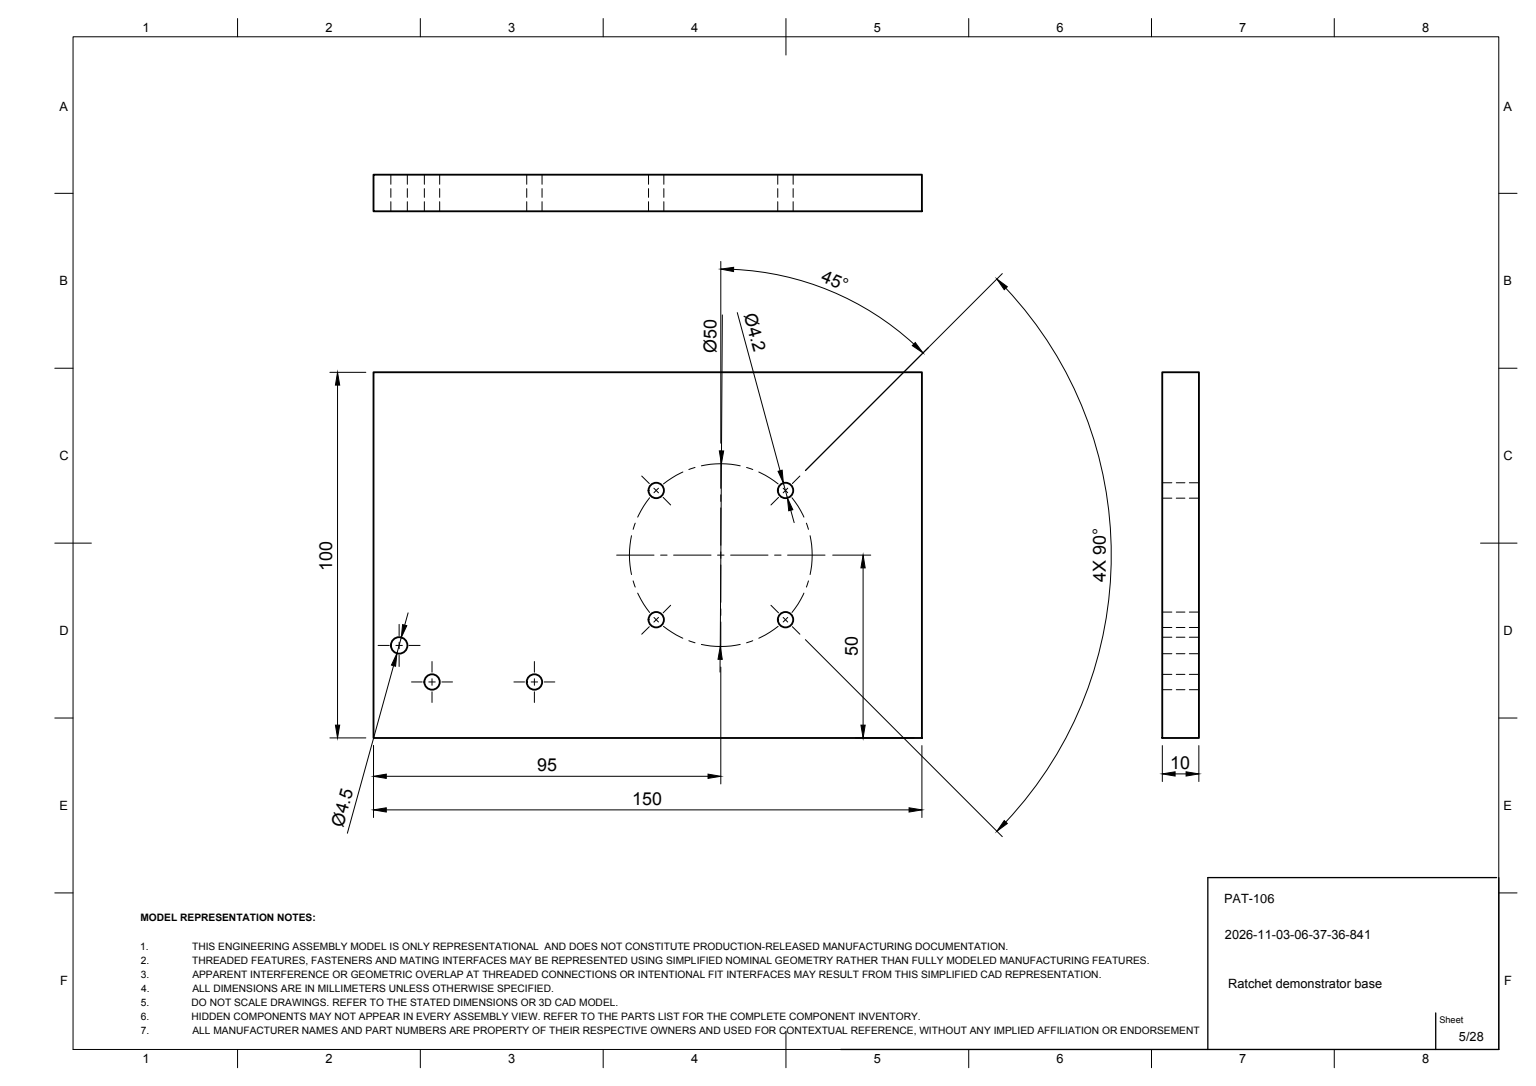
ISO-10303-21;
HEADER;
/* Generated by software containing ST-Developer
 * from STEP Tools, Inc. (www.steptools.com) 
 */

FILE_DESCRIPTION(
/* description */ ('Torsion-spring ratchet demonstrator'),
/* implementation_level */ '2;1');

FILE_NAME(
/* name */ 'Ratchet demonstrator base.step',
/* time_stamp */ '2026-10-29T17:29:17-07:00',
/* author */ (''),
/* organization */ (''),
/* preprocessor_version */ 'ST-DEVELOPER v20.2',
/* originating_system */ 'Autodesk Translation Framework v15.17.0.0',
/* authorisation */ '');

FILE_SCHEMA (('AUTOMOTIVE_DESIGN { 1 0 10303 214 3 1 1 }'));
ENDSEC;

DATA;
#10=MECHANICAL_DESIGN_GEOMETRIC_PRESENTATION_REPRESENTATION('',(#283),#11258);
#235=SHAPE_REPRESENTATION_RELATIONSHIP('SRR','None',#11361,#259);
#259=ADVANCED_BREP_SHAPE_REPRESENTATION('',(#315),#11231);
#283=STYLED_ITEM('',(#11563),#315);
#315=MANIFOLD_SOLID_BREP('Body1',#5154);
#345=FACE_BOUND('',#940,.T.);
#346=FACE_BOUND('',#941,.T.);
#347=FACE_BOUND('',#942,.T.);
#348=FACE_BOUND('',#943,.T.);
#349=FACE_BOUND('',#944,.T.);
#350=FACE_BOUND('',#945,.T.);
#351=FACE_BOUND('',#946,.T.);
#352=FACE_BOUND('',#948,.T.);
#353=FACE_BOUND('',#949,.T.);
#354=FACE_BOUND('',#950,.T.);
#355=FACE_BOUND('',#951,.T.);
#356=FACE_BOUND('',#952,.T.);
#357=FACE_BOUND('',#953,.T.);
#358=FACE_BOUND('',#954,.T.);
#437=PLANE('',#5477);
#438=PLANE('',#5478);
#439=PLANE('',#5479);
#440=PLANE('',#5480);
#441=PLANE('',#5481);
#442=PLANE('',#5482);
#623=FACE_OUTER_BOUND('',#928,.T.);
#624=FACE_OUTER_BOUND('',#929,.T.);
#625=FACE_OUTER_BOUND('',#930,.T.);
#626=FACE_OUTER_BOUND('',#931,.T.);
#627=FACE_OUTER_BOUND('',#932,.T.);
#628=FACE_OUTER_BOUND('',#933,.T.);
#629=FACE_OUTER_BOUND('',#934,.T.);
#630=FACE_OUTER_BOUND('',#935,.T.);
#631=FACE_OUTER_BOUND('',#936,.T.);
#632=FACE_OUTER_BOUND('',#937,.T.);
#633=FACE_OUTER_BOUND('',#938,.T.);
#634=FACE_OUTER_BOUND('',#939,.T.);
#635=FACE_OUTER_BOUND('',#947,.T.);
#928=EDGE_LOOP('',(#3442,#3443,#3444,#3445));
#929=EDGE_LOOP('',(#3446,#3447,#3448,#3449));
#930=EDGE_LOOP('',(#3450,#3451,#3452,#3453));
#931=EDGE_LOOP('',(#3454,#3455,#3456,#3457));
#932=EDGE_LOOP('',(#3458,#3459,#3460,#3461));
#933=EDGE_LOOP('',(#3462,#3463,#3464,#3465));
#934=EDGE_LOOP('',(#3466,#3467,#3468,#3469));
#935=EDGE_LOOP('',(#3470,#3471,#3472,#3473));
#936=EDGE_LOOP('',(#3474,#3475,#3476,#3477));
#937=EDGE_LOOP('',(#3478,#3479,#3480,#3481));
#938=EDGE_LOOP('',(#3482,#3483,#3484,#3485));
#939=EDGE_LOOP('',(#3486,#3487,#3488,#3489));
#940=EDGE_LOOP('',(#3490));
#941=EDGE_LOOP('',(#3491));
#942=EDGE_LOOP('',(#3492));
#943=EDGE_LOOP('',(#3493));
#944=EDGE_LOOP('',(#3494));
#945=EDGE_LOOP('',(#3495));
#946=EDGE_LOOP('',(#3496));
#947=EDGE_LOOP('',(#3497,#3498,#3499,#3500));
#948=EDGE_LOOP('',(#3501));
#949=EDGE_LOOP('',(#3502));
#950=EDGE_LOOP('',(#3503));
#951=EDGE_LOOP('',(#3504));
#952=EDGE_LOOP('',(#3505));
#953=EDGE_LOOP('',(#3506));
#954=EDGE_LOOP('',(#3507));
#1325=LINE('',#7682,#1708);
#1326=LINE('',#7688,#1709);
#1327=LINE('',#7694,#1710);
#1328=LINE('',#7700,#1711);
#1329=LINE('',#7706,#1712);
#1330=LINE('',#7712,#1713);
#1331=LINE('',#7718,#1714);
#1332=LINE('',#7723,#1715);
#1333=LINE('',#7725,#1716);
#1334=LINE('',#7727,#1717);
#1335=LINE('',#7728,#1718);
#1336=LINE('',#7731,#1719);
#1337=LINE('',#7733,#1720);
#1338=LINE('',#7734,#1721);
#1339=LINE('',#7737,#1722);
#1340=LINE('',#7739,#1723);
#1341=LINE('',#7740,#1724);
#1342=LINE('',#7742,#1725);
#1343=LINE('',#7743,#1726);
#1708=VECTOR('',#6076,0.225);
#1709=VECTOR('',#6083,0.210000000000001);
#1710=VECTOR('',#6090,0.21);
#1711=VECTOR('',#6097,0.21);
#1712=VECTOR('',#6104,0.21);
#1713=VECTOR('',#6111,0.21);
#1714=VECTOR('',#6118,0.21);
#1715=VECTOR('',#6123,1.);
#1716=VECTOR('',#6124,1.);
#1717=VECTOR('',#6125,1.);
#1718=VECTOR('',#6126,1.);
#1719=VECTOR('',#6129,1.);
#1720=VECTOR('',#6130,1.);
#1721=VECTOR('',#6131,1.);
#1722=VECTOR('',#6134,1.);
#1723=VECTOR('',#6135,1.);
#1724=VECTOR('',#6136,1.);
#1725=VECTOR('',#6139,1.);
#1726=VECTOR('',#6140,1.);
#2091=CIRCLE('',#5457,0.225);
#2092=CIRCLE('',#5458,0.225);
#2093=CIRCLE('',#5460,0.210000000000001);
#2094=CIRCLE('',#5461,0.210000000000001);
#2095=CIRCLE('',#5463,0.21);
#2096=CIRCLE('',#5464,0.21);
#2097=CIRCLE('',#5466,0.21);
#2098=CIRCLE('',#5467,0.21);
#2099=CIRCLE('',#5469,0.21);
#2100=CIRCLE('',#5470,0.21);
#2101=CIRCLE('',#5472,0.21);
#2102=CIRCLE('',#5473,0.21);
#2103=CIRCLE('',#5475,0.21);
#2104=CIRCLE('',#5476,0.21);
#2335=VERTEX_POINT('',#7679);
#2336=VERTEX_POINT('',#7681);
#2337=VERTEX_POINT('',#7685);
#2338=VERTEX_POINT('',#7687);
#2339=VERTEX_POINT('',#7691);
#2340=VERTEX_POINT('',#7693);
#2341=VERTEX_POINT('',#7697);
#2342=VERTEX_POINT('',#7699);
#2343=VERTEX_POINT('',#7703);
#2344=VERTEX_POINT('',#7705);
#2345=VERTEX_POINT('',#7709);
#2346=VERTEX_POINT('',#7711);
#2347=VERTEX_POINT('',#7715);
#2348=VERTEX_POINT('',#7717);
#2349=VERTEX_POINT('',#7721);
#2350=VERTEX_POINT('',#7722);
#2351=VERTEX_POINT('',#7724);
#2352=VERTEX_POINT('',#7726);
#2353=VERTEX_POINT('',#7730);
#2354=VERTEX_POINT('',#7732);
#2355=VERTEX_POINT('',#7736);
#2356=VERTEX_POINT('',#7738);
#2781=EDGE_CURVE('',#2335,#2335,#2091,.T.);
#2782=EDGE_CURVE('',#2335,#2336,#1325,.T.);
#2783=EDGE_CURVE('',#2336,#2336,#2092,.T.);
#2784=EDGE_CURVE('',#2337,#2337,#2093,.T.);
#2785=EDGE_CURVE('',#2337,#2338,#1326,.T.);
#2786=EDGE_CURVE('',#2338,#2338,#2094,.T.);
#2787=EDGE_CURVE('',#2339,#2339,#2095,.T.);
#2788=EDGE_CURVE('',#2339,#2340,#1327,.T.);
#2789=EDGE_CURVE('',#2340,#2340,#2096,.T.);
#2790=EDGE_CURVE('',#2341,#2341,#2097,.T.);
#2791=EDGE_CURVE('',#2341,#2342,#1328,.T.);
#2792=EDGE_CURVE('',#2342,#2342,#2098,.T.);
#2793=EDGE_CURVE('',#2343,#2343,#2099,.T.);
#2794=EDGE_CURVE('',#2343,#2344,#1329,.T.);
#2795=EDGE_CURVE('',#2344,#2344,#2100,.T.);
#2796=EDGE_CURVE('',#2345,#2345,#2101,.T.);
#2797=EDGE_CURVE('',#2345,#2346,#1330,.T.);
#2798=EDGE_CURVE('',#2346,#2346,#2102,.T.);
#2799=EDGE_CURVE('',#2347,#2347,#2103,.T.);
#2800=EDGE_CURVE('',#2347,#2348,#1331,.T.);
#2801=EDGE_CURVE('',#2348,#2348,#2104,.T.);
#2802=EDGE_CURVE('',#2349,#2350,#1332,.T.);
#2803=EDGE_CURVE('',#2350,#2351,#1333,.T.);
#2804=EDGE_CURVE('',#2352,#2351,#1334,.T.);
#2805=EDGE_CURVE('',#2349,#2352,#1335,.T.);
#2806=EDGE_CURVE('',#2353,#2349,#1336,.T.);
#2807=EDGE_CURVE('',#2354,#2352,#1337,.T.);
#2808=EDGE_CURVE('',#2353,#2354,#1338,.T.);
#2809=EDGE_CURVE('',#2355,#2353,#1339,.T.);
#2810=EDGE_CURVE('',#2356,#2354,#1340,.T.);
#2811=EDGE_CURVE('',#2355,#2356,#1341,.T.);
#2812=EDGE_CURVE('',#2350,#2355,#1342,.T.);
#2813=EDGE_CURVE('',#2351,#2356,#1343,.T.);
#3442=ORIENTED_EDGE('',*,*,#2781,.F.);
#3443=ORIENTED_EDGE('',*,*,#2782,.T.);
#3444=ORIENTED_EDGE('',*,*,#2783,.F.);
#3445=ORIENTED_EDGE('',*,*,#2782,.F.);
#3446=ORIENTED_EDGE('',*,*,#2784,.F.);
#3447=ORIENTED_EDGE('',*,*,#2785,.T.);
#3448=ORIENTED_EDGE('',*,*,#2786,.F.);
#3449=ORIENTED_EDGE('',*,*,#2785,.F.);
#3450=ORIENTED_EDGE('',*,*,#2787,.F.);
#3451=ORIENTED_EDGE('',*,*,#2788,.T.);
#3452=ORIENTED_EDGE('',*,*,#2789,.F.);
#3453=ORIENTED_EDGE('',*,*,#2788,.F.);
#3454=ORIENTED_EDGE('',*,*,#2790,.F.);
#3455=ORIENTED_EDGE('',*,*,#2791,.T.);
#3456=ORIENTED_EDGE('',*,*,#2792,.F.);
#3457=ORIENTED_EDGE('',*,*,#2791,.F.);
#3458=ORIENTED_EDGE('',*,*,#2793,.F.);
#3459=ORIENTED_EDGE('',*,*,#2794,.T.);
#3460=ORIENTED_EDGE('',*,*,#2795,.F.);
#3461=ORIENTED_EDGE('',*,*,#2794,.F.);
#3462=ORIENTED_EDGE('',*,*,#2796,.F.);
#3463=ORIENTED_EDGE('',*,*,#2797,.T.);
#3464=ORIENTED_EDGE('',*,*,#2798,.F.);
#3465=ORIENTED_EDGE('',*,*,#2797,.F.);
#3466=ORIENTED_EDGE('',*,*,#2799,.F.);
#3467=ORIENTED_EDGE('',*,*,#2800,.T.);
#3468=ORIENTED_EDGE('',*,*,#2801,.F.);
#3469=ORIENTED_EDGE('',*,*,#2800,.F.);
#3470=ORIENTED_EDGE('',*,*,#2802,.T.);
#3471=ORIENTED_EDGE('',*,*,#2803,.T.);
#3472=ORIENTED_EDGE('',*,*,#2804,.F.);
#3473=ORIENTED_EDGE('',*,*,#2805,.F.);
#3474=ORIENTED_EDGE('',*,*,#2806,.T.);
#3475=ORIENTED_EDGE('',*,*,#2805,.T.);
#3476=ORIENTED_EDGE('',*,*,#2807,.F.);
#3477=ORIENTED_EDGE('',*,*,#2808,.F.);
#3478=ORIENTED_EDGE('',*,*,#2809,.T.);
#3479=ORIENTED_EDGE('',*,*,#2808,.T.);
#3480=ORIENTED_EDGE('',*,*,#2810,.F.);
#3481=ORIENTED_EDGE('',*,*,#2811,.F.);
#3482=ORIENTED_EDGE('',*,*,#2812,.T.);
#3483=ORIENTED_EDGE('',*,*,#2811,.T.);
#3484=ORIENTED_EDGE('',*,*,#2813,.F.);
#3485=ORIENTED_EDGE('',*,*,#2803,.F.);
#3486=ORIENTED_EDGE('',*,*,#2813,.T.);
#3487=ORIENTED_EDGE('',*,*,#2810,.T.);
#3488=ORIENTED_EDGE('',*,*,#2807,.T.);
#3489=ORIENTED_EDGE('',*,*,#2804,.T.);
#3490=ORIENTED_EDGE('',*,*,#2783,.T.);
#3491=ORIENTED_EDGE('',*,*,#2786,.T.);
#3492=ORIENTED_EDGE('',*,*,#2789,.T.);
#3493=ORIENTED_EDGE('',*,*,#2792,.T.);
#3494=ORIENTED_EDGE('',*,*,#2795,.T.);
#3495=ORIENTED_EDGE('',*,*,#2798,.T.);
#3496=ORIENTED_EDGE('',*,*,#2801,.T.);
#3497=ORIENTED_EDGE('',*,*,#2812,.F.);
#3498=ORIENTED_EDGE('',*,*,#2802,.F.);
#3499=ORIENTED_EDGE('',*,*,#2806,.F.);
#3500=ORIENTED_EDGE('',*,*,#2809,.F.);
#3501=ORIENTED_EDGE('',*,*,#2781,.T.);
#3502=ORIENTED_EDGE('',*,*,#2784,.T.);
#3503=ORIENTED_EDGE('',*,*,#2787,.T.);
#3504=ORIENTED_EDGE('',*,*,#2790,.T.);
#3505=ORIENTED_EDGE('',*,*,#2793,.T.);
#3506=ORIENTED_EDGE('',*,*,#2796,.T.);
#3507=ORIENTED_EDGE('',*,*,#2799,.T.);
#4764=CYLINDRICAL_SURFACE('',#5456,0.225);
#4765=CYLINDRICAL_SURFACE('',#5459,0.210000000000001);
#4766=CYLINDRICAL_SURFACE('',#5462,0.21);
#4767=CYLINDRICAL_SURFACE('',#5465,0.21);
#4768=CYLINDRICAL_SURFACE('',#5468,0.21);
#4769=CYLINDRICAL_SURFACE('',#5471,0.21);
#4770=CYLINDRICAL_SURFACE('',#5474,0.21);
#4849=ADVANCED_FACE('',(#623),#4764,.F.);
#4850=ADVANCED_FACE('',(#624),#4765,.F.);
#4851=ADVANCED_FACE('',(#625),#4766,.F.);
#4852=ADVANCED_FACE('',(#626),#4767,.F.);
#4853=ADVANCED_FACE('',(#627),#4768,.F.);
#4854=ADVANCED_FACE('',(#628),#4769,.F.);
#4855=ADVANCED_FACE('',(#629),#4770,.F.);
#4856=ADVANCED_FACE('',(#630),#437,.T.);
#4857=ADVANCED_FACE('',(#631),#438,.T.);
#4858=ADVANCED_FACE('',(#632),#439,.T.);
#4859=ADVANCED_FACE('',(#633),#440,.T.);
#4860=ADVANCED_FACE('',(#634,#345,#346,#347,#348,#349,#350,#351),#441,.T.);
#4861=ADVANCED_FACE('',(#635,#352,#353,#354,#355,#356,#357,#358),#442,.F.);
#5154=CLOSED_SHELL('',(#4849,#4850,#4851,#4852,#4853,#4854,#4855,#4856,
#4857,#4858,#4859,#4860,#4861));
#5455=AXIS2_PLACEMENT_3D('',#7677,#6070,#6071);
#5456=AXIS2_PLACEMENT_3D('',#7678,#6072,#6073);
#5457=AXIS2_PLACEMENT_3D('',#7680,#6074,#6075);
#5458=AXIS2_PLACEMENT_3D('',#7683,#6077,#6078);
#5459=AXIS2_PLACEMENT_3D('',#7684,#6079,#6080);
#5460=AXIS2_PLACEMENT_3D('',#7686,#6081,#6082);
#5461=AXIS2_PLACEMENT_3D('',#7689,#6084,#6085);
#5462=AXIS2_PLACEMENT_3D('',#7690,#6086,#6087);
#5463=AXIS2_PLACEMENT_3D('',#7692,#6088,#6089);
#5464=AXIS2_PLACEMENT_3D('',#7695,#6091,#6092);
#5465=AXIS2_PLACEMENT_3D('',#7696,#6093,#6094);
#5466=AXIS2_PLACEMENT_3D('',#7698,#6095,#6096);
#5467=AXIS2_PLACEMENT_3D('',#7701,#6098,#6099);
#5468=AXIS2_PLACEMENT_3D('',#7702,#6100,#6101);
#5469=AXIS2_PLACEMENT_3D('',#7704,#6102,#6103);
#5470=AXIS2_PLACEMENT_3D('',#7707,#6105,#6106);
#5471=AXIS2_PLACEMENT_3D('',#7708,#6107,#6108);
#5472=AXIS2_PLACEMENT_3D('',#7710,#6109,#6110);
#5473=AXIS2_PLACEMENT_3D('',#7713,#6112,#6113);
#5474=AXIS2_PLACEMENT_3D('',#7714,#6114,#6115);
#5475=AXIS2_PLACEMENT_3D('',#7716,#6116,#6117);
#5476=AXIS2_PLACEMENT_3D('',#7719,#6119,#6120);
#5477=AXIS2_PLACEMENT_3D('',#7720,#6121,#6122);
#5478=AXIS2_PLACEMENT_3D('',#7729,#6127,#6128);
#5479=AXIS2_PLACEMENT_3D('',#7735,#6132,#6133);
#5480=AXIS2_PLACEMENT_3D('',#7741,#6137,#6138);
#5481=AXIS2_PLACEMENT_3D('',#7744,#6141,#6142);
#5482=AXIS2_PLACEMENT_3D('',#7745,#6143,#6144);
#6070=DIRECTION('axis',(0.,0.,1.));
#6071=DIRECTION('refdir',(1.,0.,0.));
#6072=DIRECTION('center_axis',(0.,0.,1.));
#6073=DIRECTION('ref_axis',(1.,0.,0.));
#6074=DIRECTION('center_axis',(0.,0.,1.));
#6075=DIRECTION('ref_axis',(1.,0.,0.));
#6076=DIRECTION('',(0.,0.,1.));
#6077=DIRECTION('center_axis',(0.,0.,-1.));
#6078=DIRECTION('ref_axis',(1.,0.,0.));
#6079=DIRECTION('center_axis',(0.,0.,1.));
#6080=DIRECTION('ref_axis',(1.,0.,0.));
#6081=DIRECTION('center_axis',(0.,0.,1.));
#6082=DIRECTION('ref_axis',(1.,0.,0.));
#6083=DIRECTION('',(0.,0.,1.));
#6084=DIRECTION('center_axis',(0.,0.,-1.));
#6085=DIRECTION('ref_axis',(1.,0.,0.));
#6086=DIRECTION('center_axis',(0.,0.,1.));
#6087=DIRECTION('ref_axis',(1.,0.,0.));
#6088=DIRECTION('center_axis',(0.,0.,1.));
#6089=DIRECTION('ref_axis',(1.,0.,0.));
#6090=DIRECTION('',(0.,0.,1.));
#6091=DIRECTION('center_axis',(0.,0.,-1.));
#6092=DIRECTION('ref_axis',(1.,0.,0.));
#6093=DIRECTION('center_axis',(0.,0.,1.));
#6094=DIRECTION('ref_axis',(1.,0.,0.));
#6095=DIRECTION('center_axis',(0.,0.,1.));
#6096=DIRECTION('ref_axis',(1.,0.,0.));
#6097=DIRECTION('',(0.,0.,1.));
#6098=DIRECTION('center_axis',(0.,0.,-1.));
#6099=DIRECTION('ref_axis',(1.,0.,0.));
#6100=DIRECTION('center_axis',(0.,0.,1.));
#6101=DIRECTION('ref_axis',(1.,0.,0.));
#6102=DIRECTION('center_axis',(0.,0.,1.));
#6103=DIRECTION('ref_axis',(1.,0.,0.));
#6104=DIRECTION('',(0.,0.,1.));
#6105=DIRECTION('center_axis',(0.,0.,-1.));
#6106=DIRECTION('ref_axis',(1.,0.,0.));
#6107=DIRECTION('center_axis',(0.,0.,1.));
#6108=DIRECTION('ref_axis',(1.,0.,0.));
#6109=DIRECTION('center_axis',(0.,0.,1.));
#6110=DIRECTION('ref_axis',(1.,0.,0.));
#6111=DIRECTION('',(0.,0.,1.));
#6112=DIRECTION('center_axis',(0.,0.,-1.));
#6113=DIRECTION('ref_axis',(1.,0.,0.));
#6114=DIRECTION('center_axis',(0.,0.,1.));
#6115=DIRECTION('ref_axis',(1.,0.,0.));
#6116=DIRECTION('center_axis',(0.,0.,1.));
#6117=DIRECTION('ref_axis',(1.,0.,0.));
#6118=DIRECTION('',(0.,0.,1.));
#6119=DIRECTION('center_axis',(0.,0.,-1.));
#6120=DIRECTION('ref_axis',(1.,0.,0.));
#6121=DIRECTION('center_axis',(0.,1.,0.));
#6122=DIRECTION('ref_axis',(-1.,0.,0.));
#6123=DIRECTION('',(-1.,0.,0.));
#6124=DIRECTION('',(0.,0.,1.));
#6125=DIRECTION('',(-1.,0.,0.));
#6126=DIRECTION('',(0.,0.,1.));
#6127=DIRECTION('center_axis',(1.,0.,0.));
#6128=DIRECTION('ref_axis',(0.,1.,0.));
#6129=DIRECTION('',(0.,1.,0.));
#6130=DIRECTION('',(0.,1.,0.));
#6131=DIRECTION('',(0.,0.,1.));
#6132=DIRECTION('center_axis',(0.,-1.,0.));
#6133=DIRECTION('ref_axis',(1.,0.,0.));
#6134=DIRECTION('',(1.,0.,0.));
#6135=DIRECTION('',(1.,0.,0.));
#6136=DIRECTION('',(0.,0.,1.));
#6137=DIRECTION('center_axis',(-1.,0.,0.));
#6138=DIRECTION('ref_axis',(0.,-1.,0.));
#6139=DIRECTION('',(0.,-1.,0.));
#6140=DIRECTION('',(0.,-1.,0.));
#6141=DIRECTION('center_axis',(0.,0.,1.));
#6142=DIRECTION('ref_axis',(1.,0.,0.));
#6143=DIRECTION('center_axis',(0.,0.,1.));
#6144=DIRECTION('ref_axis',(1.,0.,0.));
#7677=CARTESIAN_POINT('',(0.,0.,0.));
#7678=CARTESIAN_POINT('Origin',(8.8,-2.47,-0.1));
#7679=CARTESIAN_POINT('',(8.575,-2.47,0.));
#7680=CARTESIAN_POINT('Origin',(8.8,-2.47,0.));
#7681=CARTESIAN_POINT('',(8.575,-2.47,1.));
#7682=CARTESIAN_POINT('',(8.575,-2.47,-0.1));
#7683=CARTESIAN_POINT('Origin',(8.8,-2.47,1.));
#7684=CARTESIAN_POINT('Origin',(7.9,-3.47,-0.1));
#7685=CARTESIAN_POINT('',(7.69,-3.47,0.));
#7686=CARTESIAN_POINT('Origin',(7.9,-3.47,0.));
#7687=CARTESIAN_POINT('',(7.69,-3.47,1.));
#7688=CARTESIAN_POINT('',(7.69,-3.47,-0.1));
#7689=CARTESIAN_POINT('Origin',(7.9,-3.47,1.));
#7690=CARTESIAN_POINT('Origin',(5.1,-3.47,-0.1));
#7691=CARTESIAN_POINT('',(4.89,-3.47,0.));
#7692=CARTESIAN_POINT('Origin',(5.1,-3.47,0.));
#7693=CARTESIAN_POINT('',(4.89,-3.47,1.));
#7694=CARTESIAN_POINT('',(4.89,-3.47,-0.1));
#7695=CARTESIAN_POINT('Origin',(5.1,-3.47,1.));
#7696=CARTESIAN_POINT('Origin',(1.76776695296637,-1.76776695296637,-0.1));
#7697=CARTESIAN_POINT('',(1.55776695296637,-1.76776695296637,0.));
#7698=CARTESIAN_POINT('Origin',(1.76776695296637,-1.76776695296637,0.));
#7699=CARTESIAN_POINT('',(1.55776695296637,-1.76776695296637,1.));
#7700=CARTESIAN_POINT('',(1.55776695296637,-1.76776695296637,-0.1));
#7701=CARTESIAN_POINT('Origin',(1.76776695296637,-1.76776695296637,1.));
#7702=CARTESIAN_POINT('Origin',(-1.76776695296637,-1.76776695296637,-0.1));
#7703=CARTESIAN_POINT('',(-1.97776695296637,-1.76776695296637,0.));
#7704=CARTESIAN_POINT('Origin',(-1.76776695296637,-1.76776695296637,0.));
#7705=CARTESIAN_POINT('',(-1.97776695296637,-1.76776695296637,1.));
#7706=CARTESIAN_POINT('',(-1.97776695296637,-1.76776695296637,-0.1));
#7707=CARTESIAN_POINT('Origin',(-1.76776695296637,-1.76776695296637,1.));
#7708=CARTESIAN_POINT('Origin',(-1.76776695296637,1.76776695296637,-0.1));
#7709=CARTESIAN_POINT('',(-1.97776695296637,1.76776695296637,0.));
#7710=CARTESIAN_POINT('Origin',(-1.76776695296637,1.76776695296637,0.));
#7711=CARTESIAN_POINT('',(-1.97776695296637,1.76776695296637,1.));
#7712=CARTESIAN_POINT('',(-1.97776695296637,1.76776695296637,-0.1));
#7713=CARTESIAN_POINT('Origin',(-1.76776695296637,1.76776695296637,1.));
#7714=CARTESIAN_POINT('Origin',(1.76776695296637,1.76776695296637,-0.1));
#7715=CARTESIAN_POINT('',(1.55776695296637,1.76776695296637,0.));
#7716=CARTESIAN_POINT('Origin',(1.76776695296637,1.76776695296637,0.));
#7717=CARTESIAN_POINT('',(1.55776695296637,1.76776695296637,1.));
#7718=CARTESIAN_POINT('',(1.55776695296637,1.76776695296637,-0.1));
#7719=CARTESIAN_POINT('Origin',(1.76776695296637,1.76776695296637,1.));
#7720=CARTESIAN_POINT('Origin',(9.5,5.,0.));
#7721=CARTESIAN_POINT('',(9.5,5.,0.));
#7722=CARTESIAN_POINT('',(-5.5,5.,0.));
#7723=CARTESIAN_POINT('',(9.5,5.,0.));
#7724=CARTESIAN_POINT('',(-5.5,5.,1.));
#7725=CARTESIAN_POINT('',(-5.5,5.,0.));
#7726=CARTESIAN_POINT('',(9.5,5.,1.));
#7727=CARTESIAN_POINT('',(9.5,5.,1.));
#7728=CARTESIAN_POINT('',(9.5,5.,0.));
#7729=CARTESIAN_POINT('Origin',(9.5,-5.,0.));
#7730=CARTESIAN_POINT('',(9.5,-5.,0.));
#7731=CARTESIAN_POINT('',(9.5,-5.,0.));
#7732=CARTESIAN_POINT('',(9.5,-5.,1.));
#7733=CARTESIAN_POINT('',(9.5,-5.,1.));
#7734=CARTESIAN_POINT('',(9.5,-5.,0.));
#7735=CARTESIAN_POINT('Origin',(-5.5,-5.,0.));
#7736=CARTESIAN_POINT('',(-5.5,-5.,0.));
#7737=CARTESIAN_POINT('',(-5.5,-5.,0.));
#7738=CARTESIAN_POINT('',(-5.5,-5.,1.));
#7739=CARTESIAN_POINT('',(-5.5,-5.,1.));
#7740=CARTESIAN_POINT('',(-5.5,-5.,0.));
#7741=CARTESIAN_POINT('Origin',(-5.5,5.,0.));
#7742=CARTESIAN_POINT('',(-5.5,5.,0.));
#7743=CARTESIAN_POINT('',(-5.5,5.,1.));
#7744=CARTESIAN_POINT('Origin',(2.,0.,1.));
#7745=CARTESIAN_POINT('Origin',(2.,0.,0.));
#11201=UNCERTAINTY_MEASURE_WITH_UNIT(LENGTH_MEASURE(0.001),#11259,
'DISTANCE_ACCURACY_VALUE',
'Maximum model space distance between geometric entities at asserted c
onnectivities');
#11228=UNCERTAINTY_MEASURE_WITH_UNIT(LENGTH_MEASURE(0.001),#11259,
'DISTANCE_ACCURACY_VALUE',
'Maximum model space distance between geometric entities at asserted c
onnectivities');
#11231=(
GEOMETRIC_REPRESENTATION_CONTEXT(3)
GLOBAL_UNCERTAINTY_ASSIGNED_CONTEXT((#11201))
GLOBAL_UNIT_ASSIGNED_CONTEXT((#11259,#11261,#11262))
REPRESENTATION_CONTEXT('','3D')
);
#11258=(
GEOMETRIC_REPRESENTATION_CONTEXT(3)
GLOBAL_UNCERTAINTY_ASSIGNED_CONTEXT((#11228))
GLOBAL_UNIT_ASSIGNED_CONTEXT((#11259,#11261,#11262))
REPRESENTATION_CONTEXT('','3D')
);
#11259=(
LENGTH_UNIT()
NAMED_UNIT(*)
SI_UNIT(.CENTI.,.METRE.)
);
#11261=(
NAMED_UNIT(*)
PLANE_ANGLE_UNIT()
SI_UNIT($,.RADIAN.)
);
#11262=(
NAMED_UNIT(*)
SI_UNIT($,.STERADIAN.)
SOLID_ANGLE_UNIT()
);
#11265=SHAPE_DEFINITION_REPRESENTATION(#11294,#11361);
#11294=PRODUCT_DEFINITION_SHAPE('',$,#11391);
#11361=SHAPE_REPRESENTATION('',(#5455),#11231);
#11388=PRODUCT_DEFINITION_CONTEXT('part definition',#11477,'design');
#11391=PRODUCT_DEFINITION('Ratchet demonstrator base',
'Ratchet demonstrator base',#11420,#11388);
#11420=PRODUCT_DEFINITION_FORMATION('',$,#11481);
#11477=APPLICATION_CONTEXT(
'Core Data for Automotive Mechanical Design Process');
#11478=PRODUCT_CONTEXT('part definition',#11477,'mechanical');
#11481=PRODUCT('Ratchet demonstrator base','Ratchet demonstrator base',
'Ratchet demonstrator base',(#11478));
#11557=COLOUR_RGB('Dark Blue',0.08,0.2,0.34);
#11558=FILL_AREA_STYLE_COLOUR('',#11557);
#11559=FILL_AREA_STYLE('',(#11558));
#11560=SURFACE_STYLE_FILL_AREA(#11559);
#11561=SURFACE_SIDE_STYLE('',(#11560));
#11562=SURFACE_STYLE_USAGE(.BOTH.,#11561);
#11563=PRESENTATION_STYLE_ASSIGNMENT((#11562));
ENDSEC;
END-ISO-10303-21;
